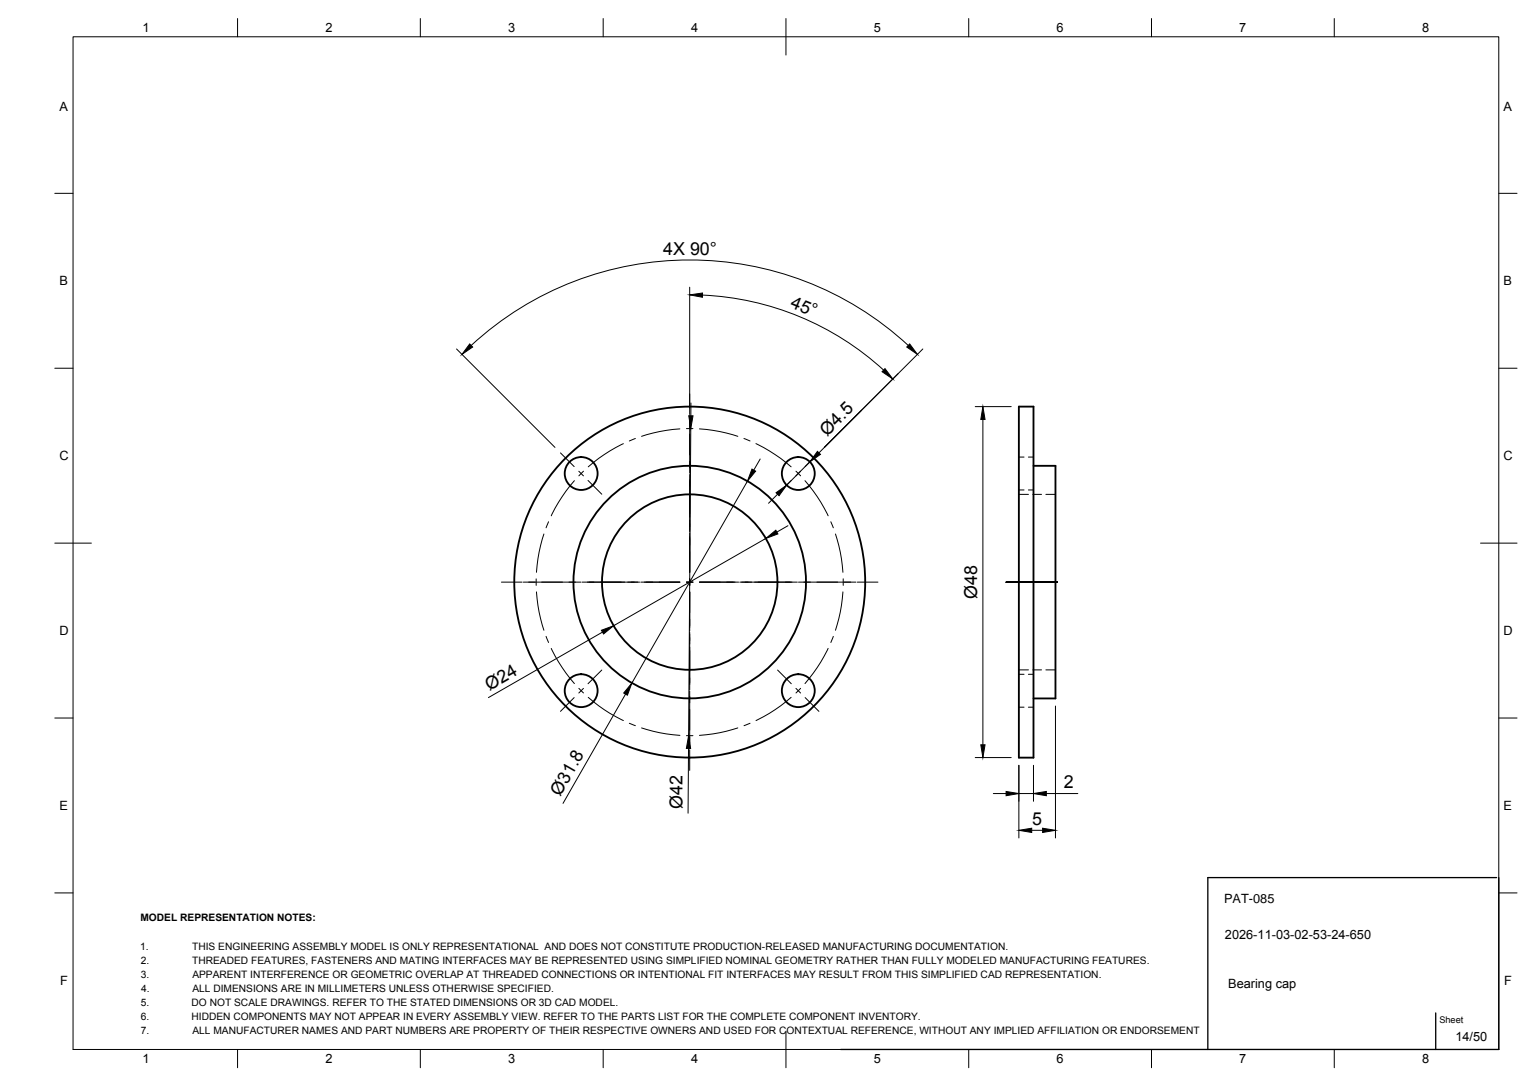
ISO-10303-21;
HEADER;
/* Generated by software containing ST-Developer
 * from STEP Tools, Inc. (www.steptools.com) 
 */

FILE_DESCRIPTION(
/* description */ ('Rack and pinion manual slide'),
/* implementation_level */ '2;1');

FILE_NAME(
/* name */ 'Bearing cap.step',
/* time_stamp */ '2026-10-28T03:22:49-07:00',
/* author */ (''),
/* organization */ (''),
/* preprocessor_version */ 'ST-DEVELOPER v20.2',
/* originating_system */ 'Autodesk Translation Framework v15.17.0.0',
/* authorisation */ '');

FILE_SCHEMA (('AUTOMOTIVE_DESIGN { 1 0 10303 214 3 1 1 }'));
ENDSEC;

DATA;
#10=MECHANICAL_DESIGN_GEOMETRIC_PRESENTATION_REPRESENTATION('',(#741),#34851);
#649=SHAPE_REPRESENTATION_RELATIONSHIP('SRR','None',#35084,#695);
#695=ADVANCED_BREP_SHAPE_REPRESENTATION('',(#794),#34809);
#741=STYLED_ITEM('',(#35411),#794);
#794=MANIFOLD_SOLID_BREP('Body1',#13761);
#899=FACE_BOUND('',#2443,.T.);
#900=FACE_BOUND('',#2447,.T.);
#901=FACE_BOUND('',#2448,.T.);
#902=FACE_BOUND('',#2449,.T.);
#903=FACE_BOUND('',#2450,.T.);
#904=FACE_BOUND('',#2451,.T.);
#905=FACE_BOUND('',#2453,.T.);
#906=FACE_BOUND('',#2454,.T.);
#907=FACE_BOUND('',#2455,.T.);
#908=FACE_BOUND('',#2456,.T.);
#909=FACE_BOUND('',#2457,.T.);
#1106=PLANE('',#14511);
#1107=PLANE('',#14518);
#1108=PLANE('',#14519);
#1632=FACE_OUTER_BOUND('',#2437,.T.);
#1633=FACE_OUTER_BOUND('',#2438,.T.);
#1634=FACE_OUTER_BOUND('',#2439,.T.);
#1635=FACE_OUTER_BOUND('',#2440,.T.);
#1636=FACE_OUTER_BOUND('',#2441,.T.);
#1637=FACE_OUTER_BOUND('',#2442,.T.);
#1638=FACE_OUTER_BOUND('',#2444,.T.);
#1639=FACE_OUTER_BOUND('',#2445,.T.);
#1640=FACE_OUTER_BOUND('',#2446,.T.);
#1641=FACE_OUTER_BOUND('',#2452,.T.);
#2437=EDGE_LOOP('',(#9684,#9685,#9686,#9687));
#2438=EDGE_LOOP('',(#9688,#9689,#9690,#9691));
#2439=EDGE_LOOP('',(#9692,#9693,#9694,#9695));
#2440=EDGE_LOOP('',(#9696,#9697,#9698,#9699));
#2441=EDGE_LOOP('',(#9700,#9701,#9702,#9703));
#2442=EDGE_LOOP('',(#9704));
#2443=EDGE_LOOP('',(#9705));
#2444=EDGE_LOOP('',(#9706,#9707,#9708,#9709));
#2445=EDGE_LOOP('',(#9710,#9711,#9712,#9713));
#2446=EDGE_LOOP('',(#9714));
#2447=EDGE_LOOP('',(#9715));
#2448=EDGE_LOOP('',(#9716));
#2449=EDGE_LOOP('',(#9717));
#2450=EDGE_LOOP('',(#9718));
#2451=EDGE_LOOP('',(#9719));
#2452=EDGE_LOOP('',(#9720));
#2453=EDGE_LOOP('',(#9721));
#2454=EDGE_LOOP('',(#9722));
#2455=EDGE_LOOP('',(#9723));
#2456=EDGE_LOOP('',(#9724));
#2457=EDGE_LOOP('',(#9725));
#3379=LINE('',#19945,#4670);
#3380=LINE('',#19951,#4671);
#3381=LINE('',#19957,#4672);
#3382=LINE('',#19963,#4673);
#3383=LINE('',#19969,#4674);
#3384=LINE('',#19976,#4675);
#3385=LINE('',#19982,#4676);
#4670=VECTOR('',#16117,0.225);
#4671=VECTOR('',#16124,0.225);
#4672=VECTOR('',#16131,0.225);
#4673=VECTOR('',#16138,0.225);
#4674=VECTOR('',#16145,1.59);
#4675=VECTOR('',#16154,1.2);
#4676=VECTOR('',#16161,2.4);
#5876=CIRCLE('',#14497,0.225);
#5877=CIRCLE('',#14498,0.225);
#5878=CIRCLE('',#14500,0.225);
#5879=CIRCLE('',#14501,0.225);
#5880=CIRCLE('',#14503,0.225);
#5881=CIRCLE('',#14504,0.225);
#5882=CIRCLE('',#14506,0.225);
#5883=CIRCLE('',#14507,0.225);
#5884=CIRCLE('',#14509,1.59);
#5885=CIRCLE('',#14510,1.59);
#5886=CIRCLE('',#14512,1.2);
#5887=CIRCLE('',#14514,1.2);
#5888=CIRCLE('',#14516,2.4);
#5889=CIRCLE('',#14517,2.4);
#6374=VERTEX_POINT('',#19942);
#6375=VERTEX_POINT('',#19944);
#6376=VERTEX_POINT('',#19948);
#6377=VERTEX_POINT('',#19950);
#6378=VERTEX_POINT('',#19954);
#6379=VERTEX_POINT('',#19956);
#6380=VERTEX_POINT('',#19960);
#6381=VERTEX_POINT('',#19962);
#6382=VERTEX_POINT('',#19966);
#6383=VERTEX_POINT('',#19968);
#6384=VERTEX_POINT('',#19972);
#6385=VERTEX_POINT('',#19975);
#6386=VERTEX_POINT('',#19979);
#6387=VERTEX_POINT('',#19981);
#7654=EDGE_CURVE('',#6374,#6374,#5876,.T.);
#7655=EDGE_CURVE('',#6374,#6375,#3379,.T.);
#7656=EDGE_CURVE('',#6375,#6375,#5877,.T.);
#7657=EDGE_CURVE('',#6376,#6376,#5878,.T.);
#7658=EDGE_CURVE('',#6376,#6377,#3380,.T.);
#7659=EDGE_CURVE('',#6377,#6377,#5879,.T.);
#7660=EDGE_CURVE('',#6378,#6378,#5880,.T.);
#7661=EDGE_CURVE('',#6378,#6379,#3381,.T.);
#7662=EDGE_CURVE('',#6379,#6379,#5881,.T.);
#7663=EDGE_CURVE('',#6380,#6380,#5882,.T.);
#7664=EDGE_CURVE('',#6380,#6381,#3382,.T.);
#7665=EDGE_CURVE('',#6381,#6381,#5883,.T.);
#7666=EDGE_CURVE('',#6382,#6382,#5884,.T.);
#7667=EDGE_CURVE('',#6382,#6383,#3383,.T.);
#7668=EDGE_CURVE('',#6383,#6383,#5885,.T.);
#7669=EDGE_CURVE('',#6384,#6384,#5886,.T.);
#7670=EDGE_CURVE('',#6384,#6385,#3384,.T.);
#7671=EDGE_CURVE('',#6385,#6385,#5887,.T.);
#7672=EDGE_CURVE('',#6386,#6386,#5888,.T.);
#7673=EDGE_CURVE('',#6386,#6387,#3385,.T.);
#7674=EDGE_CURVE('',#6387,#6387,#5889,.T.);
#9684=ORIENTED_EDGE('',*,*,#7654,.F.);
#9685=ORIENTED_EDGE('',*,*,#7655,.T.);
#9686=ORIENTED_EDGE('',*,*,#7656,.F.);
#9687=ORIENTED_EDGE('',*,*,#7655,.F.);
#9688=ORIENTED_EDGE('',*,*,#7657,.F.);
#9689=ORIENTED_EDGE('',*,*,#7658,.T.);
#9690=ORIENTED_EDGE('',*,*,#7659,.F.);
#9691=ORIENTED_EDGE('',*,*,#7658,.F.);
#9692=ORIENTED_EDGE('',*,*,#7660,.F.);
#9693=ORIENTED_EDGE('',*,*,#7661,.T.);
#9694=ORIENTED_EDGE('',*,*,#7662,.F.);
#9695=ORIENTED_EDGE('',*,*,#7661,.F.);
#9696=ORIENTED_EDGE('',*,*,#7663,.F.);
#9697=ORIENTED_EDGE('',*,*,#7664,.T.);
#9698=ORIENTED_EDGE('',*,*,#7665,.F.);
#9699=ORIENTED_EDGE('',*,*,#7664,.F.);
#9700=ORIENTED_EDGE('',*,*,#7666,.F.);
#9701=ORIENTED_EDGE('',*,*,#7667,.T.);
#9702=ORIENTED_EDGE('',*,*,#7668,.F.);
#9703=ORIENTED_EDGE('',*,*,#7667,.F.);
#9704=ORIENTED_EDGE('',*,*,#7666,.T.);
#9705=ORIENTED_EDGE('',*,*,#7669,.T.);
#9706=ORIENTED_EDGE('',*,*,#7669,.F.);
#9707=ORIENTED_EDGE('',*,*,#7670,.T.);
#9708=ORIENTED_EDGE('',*,*,#7671,.T.);
#9709=ORIENTED_EDGE('',*,*,#7670,.F.);
#9710=ORIENTED_EDGE('',*,*,#7672,.F.);
#9711=ORIENTED_EDGE('',*,*,#7673,.T.);
#9712=ORIENTED_EDGE('',*,*,#7674,.T.);
#9713=ORIENTED_EDGE('',*,*,#7673,.F.);
#9714=ORIENTED_EDGE('',*,*,#7672,.T.);
#9715=ORIENTED_EDGE('',*,*,#7668,.T.);
#9716=ORIENTED_EDGE('',*,*,#7665,.T.);
#9717=ORIENTED_EDGE('',*,*,#7662,.T.);
#9718=ORIENTED_EDGE('',*,*,#7659,.T.);
#9719=ORIENTED_EDGE('',*,*,#7656,.T.);
#9720=ORIENTED_EDGE('',*,*,#7674,.F.);
#9721=ORIENTED_EDGE('',*,*,#7671,.F.);
#9722=ORIENTED_EDGE('',*,*,#7663,.T.);
#9723=ORIENTED_EDGE('',*,*,#7660,.T.);
#9724=ORIENTED_EDGE('',*,*,#7657,.T.);
#9725=ORIENTED_EDGE('',*,*,#7654,.T.);
#12879=CYLINDRICAL_SURFACE('',#14496,0.225);
#12880=CYLINDRICAL_SURFACE('',#14499,0.225);
#12881=CYLINDRICAL_SURFACE('',#14502,0.225);
#12882=CYLINDRICAL_SURFACE('',#14505,0.225);
#12883=CYLINDRICAL_SURFACE('',#14508,1.59);
#12884=CYLINDRICAL_SURFACE('',#14513,1.2);
#12885=CYLINDRICAL_SURFACE('',#14515,2.4);
#13110=ADVANCED_FACE('',(#1632),#12879,.F.);
#13111=ADVANCED_FACE('',(#1633),#12880,.F.);
#13112=ADVANCED_FACE('',(#1634),#12881,.F.);
#13113=ADVANCED_FACE('',(#1635),#12882,.F.);
#13114=ADVANCED_FACE('',(#1636),#12883,.T.);
#13115=ADVANCED_FACE('',(#1637,#899),#1106,.T.);
#13116=ADVANCED_FACE('',(#1638),#12884,.F.);
#13117=ADVANCED_FACE('',(#1639),#12885,.T.);
#13118=ADVANCED_FACE('',(#1640,#900,#901,#902,#903,#904),#1107,.T.);
#13119=ADVANCED_FACE('',(#1641,#905,#906,#907,#908,#909),#1108,.F.);
#13761=CLOSED_SHELL('',(#13110,#13111,#13112,#13113,#13114,#13115,#13116,
#13117,#13118,#13119));
#14495=AXIS2_PLACEMENT_3D('',#19940,#16111,#16112);
#14496=AXIS2_PLACEMENT_3D('',#19941,#16113,#16114);
#14497=AXIS2_PLACEMENT_3D('',#19943,#16115,#16116);
#14498=AXIS2_PLACEMENT_3D('',#19946,#16118,#16119);
#14499=AXIS2_PLACEMENT_3D('',#19947,#16120,#16121);
#14500=AXIS2_PLACEMENT_3D('',#19949,#16122,#16123);
#14501=AXIS2_PLACEMENT_3D('',#19952,#16125,#16126);
#14502=AXIS2_PLACEMENT_3D('',#19953,#16127,#16128);
#14503=AXIS2_PLACEMENT_3D('',#19955,#16129,#16130);
#14504=AXIS2_PLACEMENT_3D('',#19958,#16132,#16133);
#14505=AXIS2_PLACEMENT_3D('',#19959,#16134,#16135);
#14506=AXIS2_PLACEMENT_3D('',#19961,#16136,#16137);
#14507=AXIS2_PLACEMENT_3D('',#19964,#16139,#16140);
#14508=AXIS2_PLACEMENT_3D('',#19965,#16141,#16142);
#14509=AXIS2_PLACEMENT_3D('',#19967,#16143,#16144);
#14510=AXIS2_PLACEMENT_3D('',#19970,#16146,#16147);
#14511=AXIS2_PLACEMENT_3D('',#19971,#16148,#16149);
#14512=AXIS2_PLACEMENT_3D('',#19973,#16150,#16151);
#14513=AXIS2_PLACEMENT_3D('',#19974,#16152,#16153);
#14514=AXIS2_PLACEMENT_3D('',#19977,#16155,#16156);
#14515=AXIS2_PLACEMENT_3D('',#19978,#16157,#16158);
#14516=AXIS2_PLACEMENT_3D('',#19980,#16159,#16160);
#14517=AXIS2_PLACEMENT_3D('',#19983,#16162,#16163);
#14518=AXIS2_PLACEMENT_3D('',#19984,#16164,#16165);
#14519=AXIS2_PLACEMENT_3D('',#19985,#16166,#16167);
#16111=DIRECTION('axis',(0.,0.,1.));
#16112=DIRECTION('refdir',(1.,0.,0.));
#16113=DIRECTION('center_axis',(0.,1.,0.));
#16114=DIRECTION('ref_axis',(1.,0.,0.));
#16115=DIRECTION('center_axis',(0.,1.,0.));
#16116=DIRECTION('ref_axis',(1.,0.,0.));
#16117=DIRECTION('',(0.,1.,0.));
#16118=DIRECTION('center_axis',(0.,-1.,0.));
#16119=DIRECTION('ref_axis',(1.,0.,0.));
#16120=DIRECTION('center_axis',(0.,1.,0.));
#16121=DIRECTION('ref_axis',(1.,0.,0.));
#16122=DIRECTION('center_axis',(0.,1.,0.));
#16123=DIRECTION('ref_axis',(1.,0.,0.));
#16124=DIRECTION('',(0.,1.,0.));
#16125=DIRECTION('center_axis',(0.,-1.,0.));
#16126=DIRECTION('ref_axis',(1.,0.,0.));
#16127=DIRECTION('center_axis',(0.,1.,0.));
#16128=DIRECTION('ref_axis',(1.,0.,0.));
#16129=DIRECTION('center_axis',(0.,1.,0.));
#16130=DIRECTION('ref_axis',(1.,0.,0.));
#16131=DIRECTION('',(0.,1.,0.));
#16132=DIRECTION('center_axis',(0.,-1.,0.));
#16133=DIRECTION('ref_axis',(1.,0.,0.));
#16134=DIRECTION('center_axis',(0.,1.,0.));
#16135=DIRECTION('ref_axis',(1.,0.,0.));
#16136=DIRECTION('center_axis',(0.,1.,0.));
#16137=DIRECTION('ref_axis',(1.,0.,0.));
#16138=DIRECTION('',(0.,1.,0.));
#16139=DIRECTION('center_axis',(0.,-1.,0.));
#16140=DIRECTION('ref_axis',(1.,0.,0.));
#16141=DIRECTION('center_axis',(0.,1.,0.));
#16142=DIRECTION('ref_axis',(1.,0.,0.));
#16143=DIRECTION('center_axis',(0.,1.,0.));
#16144=DIRECTION('ref_axis',(1.,0.,0.));
#16145=DIRECTION('',(0.,-1.,0.));
#16146=DIRECTION('center_axis',(0.,-1.,0.));
#16147=DIRECTION('ref_axis',(1.,0.,0.));
#16148=DIRECTION('center_axis',(0.,1.,0.));
#16149=DIRECTION('ref_axis',(1.,0.,0.));
#16150=DIRECTION('center_axis',(0.,-1.,0.));
#16151=DIRECTION('ref_axis',(1.,0.,0.));
#16152=DIRECTION('center_axis',(0.,1.,0.));
#16153=DIRECTION('ref_axis',(1.,0.,0.));
#16154=DIRECTION('',(0.,-1.,0.));
#16155=DIRECTION('center_axis',(0.,-1.,0.));
#16156=DIRECTION('ref_axis',(1.,0.,0.));
#16157=DIRECTION('center_axis',(0.,1.,0.));
#16158=DIRECTION('ref_axis',(1.,0.,0.));
#16159=DIRECTION('center_axis',(0.,1.,0.));
#16160=DIRECTION('ref_axis',(1.,0.,0.));
#16161=DIRECTION('',(0.,-1.,0.));
#16162=DIRECTION('center_axis',(0.,1.,0.));
#16163=DIRECTION('ref_axis',(1.,0.,0.));
#16164=DIRECTION('center_axis',(0.,1.,0.));
#16165=DIRECTION('ref_axis',(1.,0.,0.));
#16166=DIRECTION('center_axis',(0.,1.,0.));
#16167=DIRECTION('ref_axis',(1.,0.,0.));
#19940=CARTESIAN_POINT('',(0.,0.,0.));
#19941=CARTESIAN_POINT('Origin',(9.51507575950825,-5.3,8.76507575950825));
#19942=CARTESIAN_POINT('',(9.29007575950825,-5.2,8.76507575950825));
#19943=CARTESIAN_POINT('Origin',(9.51507575950825,-5.2,8.76507575950825));
#19944=CARTESIAN_POINT('',(9.29007575950825,-5.,8.76507575950825));
#19945=CARTESIAN_POINT('',(9.29007575950825,-5.3,8.76507575950825));
#19946=CARTESIAN_POINT('Origin',(9.51507575950825,-5.,8.76507575950825));
#19947=CARTESIAN_POINT('Origin',(9.51507575950825,-5.3,11.7349242404918));
#19948=CARTESIAN_POINT('',(9.29007575950825,-5.2,11.7349242404918));
#19949=CARTESIAN_POINT('Origin',(9.51507575950825,-5.2,11.7349242404918));
#19950=CARTESIAN_POINT('',(9.29007575950825,-5.,11.7349242404918));
#19951=CARTESIAN_POINT('',(9.29007575950825,-5.3,11.7349242404918));
#19952=CARTESIAN_POINT('Origin',(9.51507575950825,-5.,11.7349242404918));
#19953=CARTESIAN_POINT('Origin',(12.4849242404918,-5.3,11.7349242404918));
#19954=CARTESIAN_POINT('',(12.2599242404918,-5.2,11.7349242404918));
#19955=CARTESIAN_POINT('Origin',(12.4849242404918,-5.2,11.7349242404918));
#19956=CARTESIAN_POINT('',(12.2599242404918,-5.,11.7349242404918));
#19957=CARTESIAN_POINT('',(12.2599242404918,-5.3,11.7349242404918));
#19958=CARTESIAN_POINT('Origin',(12.4849242404918,-5.,11.7349242404918));
#19959=CARTESIAN_POINT('Origin',(12.4849242404917,-5.3,8.76507575950825));
#19960=CARTESIAN_POINT('',(12.2599242404917,-5.2,8.76507575950825));
#19961=CARTESIAN_POINT('Origin',(12.4849242404917,-5.2,8.76507575950825));
#19962=CARTESIAN_POINT('',(12.2599242404917,-5.,8.76507575950825));
#19963=CARTESIAN_POINT('',(12.2599242404917,-5.3,8.76507575950825));
#19964=CARTESIAN_POINT('Origin',(12.4849242404917,-5.,8.76507575950825));
#19965=CARTESIAN_POINT('Origin',(11.,-5.,10.25));
#19966=CARTESIAN_POINT('',(9.41,-4.7,10.25));
#19967=CARTESIAN_POINT('Origin',(11.,-4.7,10.25));
#19968=CARTESIAN_POINT('',(9.41,-5.,10.25));
#19969=CARTESIAN_POINT('',(9.41,-5.,10.25));
#19970=CARTESIAN_POINT('Origin',(11.,-5.,10.25));
#19971=CARTESIAN_POINT('Origin',(11.,-4.7,10.25));
#19972=CARTESIAN_POINT('',(9.8,-4.7,10.25));
#19973=CARTESIAN_POINT('Origin',(11.,-4.7,10.25));
#19974=CARTESIAN_POINT('Origin',(11.,-5.2,10.25));
#19975=CARTESIAN_POINT('',(9.8,-5.2,10.25));
#19976=CARTESIAN_POINT('',(9.8,-5.2,10.25));
#19977=CARTESIAN_POINT('Origin',(11.,-5.2,10.25));
#19978=CARTESIAN_POINT('Origin',(11.,-5.2,10.25));
#19979=CARTESIAN_POINT('',(8.6,-5.,10.25));
#19980=CARTESIAN_POINT('Origin',(11.,-5.,10.25));
#19981=CARTESIAN_POINT('',(8.6,-5.2,10.25));
#19982=CARTESIAN_POINT('',(8.6,-5.2,10.25));
#19983=CARTESIAN_POINT('Origin',(11.,-5.2,10.25));
#19984=CARTESIAN_POINT('Origin',(11.,-5.,10.25));
#19985=CARTESIAN_POINT('Origin',(11.,-5.2,10.25));
#34755=UNCERTAINTY_MEASURE_WITH_UNIT(LENGTH_MEASURE(0.001),#34852,
'DISTANCE_ACCURACY_VALUE',
'Maximum model space distance between geometric entities at asserted c
onnectivities');
#34797=UNCERTAINTY_MEASURE_WITH_UNIT(LENGTH_MEASURE(0.001),#34852,
'DISTANCE_ACCURACY_VALUE',
'Maximum model space distance between geometric entities at asserted c
onnectivities');
#34809=(
GEOMETRIC_REPRESENTATION_CONTEXT(3)
GLOBAL_UNCERTAINTY_ASSIGNED_CONTEXT((#34755))
GLOBAL_UNIT_ASSIGNED_CONTEXT((#34852,#34854,#34855))
REPRESENTATION_CONTEXT('','3D')
);
#34851=(
GEOMETRIC_REPRESENTATION_CONTEXT(3)
GLOBAL_UNCERTAINTY_ASSIGNED_CONTEXT((#34797))
GLOBAL_UNIT_ASSIGNED_CONTEXT((#34852,#34854,#34855))
REPRESENTATION_CONTEXT('','3D')
);
#34852=(
LENGTH_UNIT()
NAMED_UNIT(*)
SI_UNIT(.CENTI.,.METRE.)
);
#34854=(
NAMED_UNIT(*)
PLANE_ANGLE_UNIT()
SI_UNIT($,.RADIAN.)
);
#34855=(
NAMED_UNIT(*)
SI_UNIT($,.STERADIAN.)
SOLID_ANGLE_UNIT()
);
#34867=SHAPE_DEFINITION_REPRESENTATION(#34920,#35084);
#34920=PRODUCT_DEFINITION_SHAPE('',$,#35138);
#35084=SHAPE_REPRESENTATION('',(#14495),#34809);
#35126=PRODUCT_DEFINITION_CONTEXT('part definition',#35287,'design');
#35138=PRODUCT_DEFINITION('Bearing cap','Bearing cap',#35191,#35126);
#35191=PRODUCT_DEFINITION_FORMATION('',$,#35300);
#35287=APPLICATION_CONTEXT(
'Core Data for Automotive Mechanical Design Process');
#35288=PRODUCT_CONTEXT('part definition',#35287,'mechanical');
#35300=PRODUCT('Bearing cap','Bearing cap','Bearing cap',(#35288));
#35405=COLOUR_RGB('Grey',0.48,0.52,0.57);
#35406=FILL_AREA_STYLE_COLOUR('',#35405);
#35407=FILL_AREA_STYLE('',(#35406));
#35408=SURFACE_STYLE_FILL_AREA(#35407);
#35409=SURFACE_SIDE_STYLE('',(#35408));
#35410=SURFACE_STYLE_USAGE(.BOTH.,#35409);
#35411=PRESENTATION_STYLE_ASSIGNMENT((#35410));
ENDSEC;
END-ISO-10303-21;
